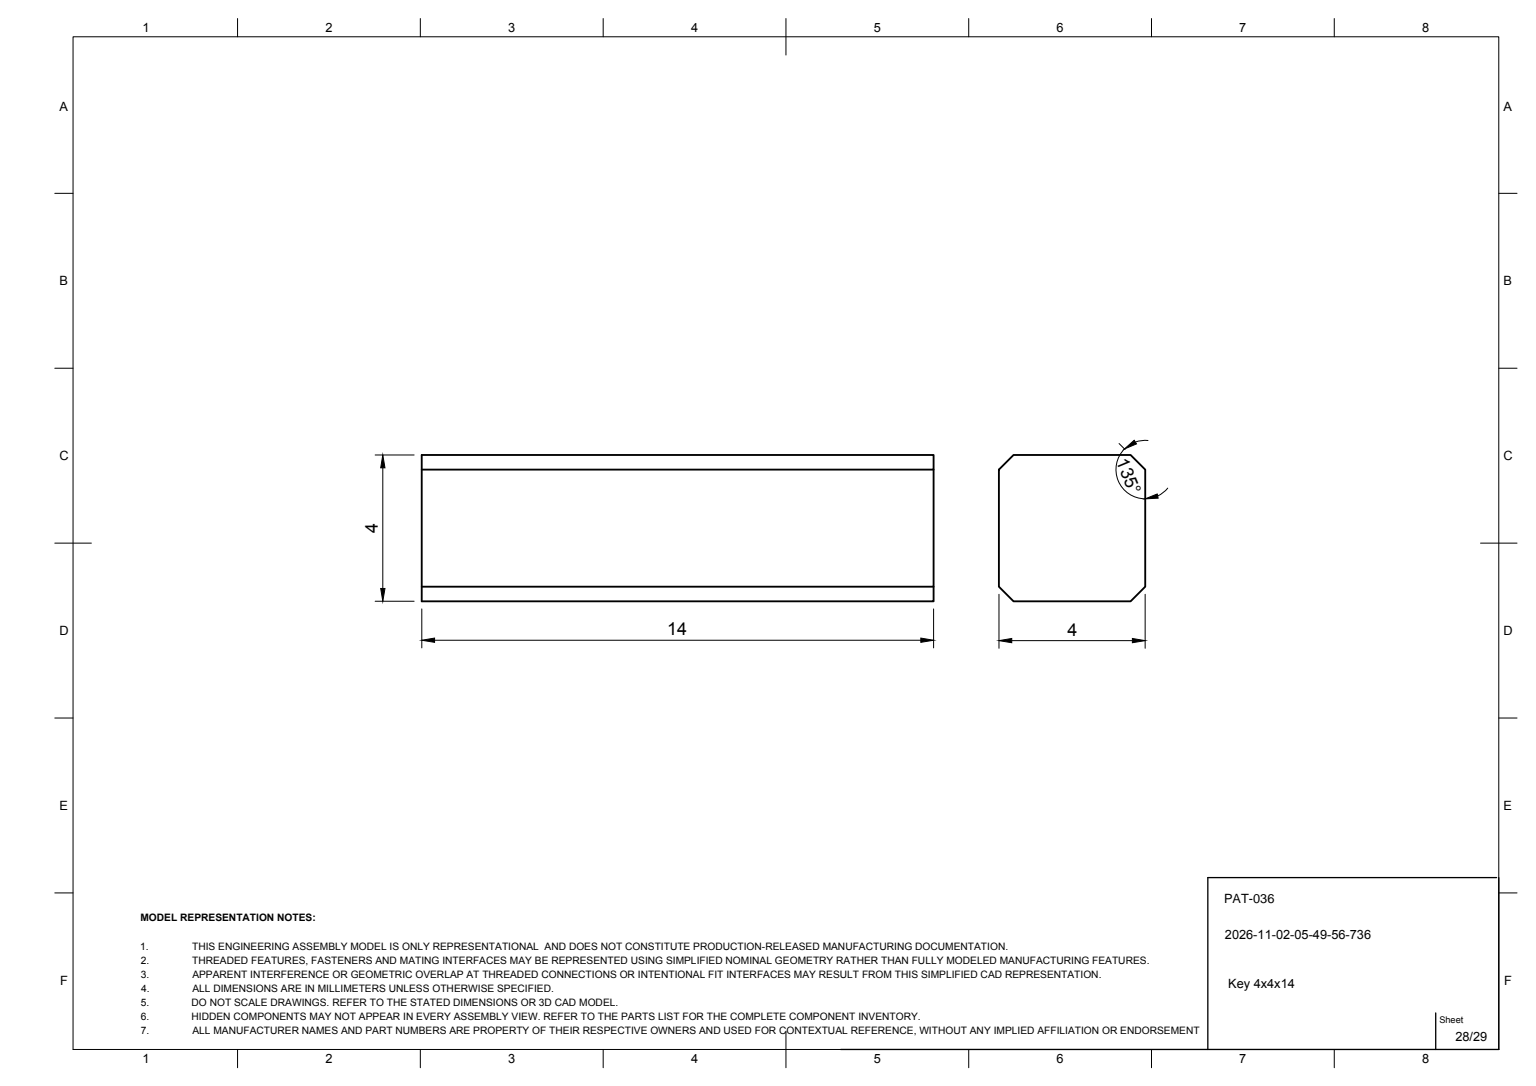
ISO-10303-21;
HEADER;
/* Generated by software containing ST-Developer
 * from STEP Tools, Inc. (www.steptools.com) 
 */

FILE_DESCRIPTION(
/* description */ ('Flange-mounted spindle'),
/* implementation_level */ '2;1');

FILE_NAME(
/* name */ 'Key 4x4x14.step',
/* time_stamp */ '2026-10-27T10:49:51-07:00',
/* author */ (''),
/* organization */ (''),
/* preprocessor_version */ 'ST-DEVELOPER v20.2',
/* originating_system */ 'Autodesk Translation Framework v15.17.0.0',
/* authorisation */ '');

FILE_SCHEMA (('AUTOMOTIVE_DESIGN { 1 0 10303 214 3 1 1 }'));
ENDSEC;

DATA;
#10=MECHANICAL_DESIGN_GEOMETRIC_PRESENTATION_REPRESENTATION('',(#360),#11764);
#305=SHAPE_REPRESENTATION_RELATIONSHIP('SRR','None',#11903,#332);
#332=ADVANCED_BREP_SHAPE_REPRESENTATION('',(#386),#11758);
#360=STYLED_ITEM('',(#12099),#386);
#386=MANIFOLD_SOLID_BREP('Body1',#6154);
#624=PLANE('',#7074);
#625=PLANE('',#7075);
#626=PLANE('',#7076);
#627=PLANE('',#7077);
#628=PLANE('',#7078);
#629=PLANE('',#7079);
#630=PLANE('',#7080);
#631=PLANE('',#7081);
#632=PLANE('',#7082);
#633=PLANE('',#7083);
#955=FACE_OUTER_BOUND('',#1409,.T.);
#956=FACE_OUTER_BOUND('',#1410,.T.);
#957=FACE_OUTER_BOUND('',#1411,.T.);
#958=FACE_OUTER_BOUND('',#1412,.T.);
#959=FACE_OUTER_BOUND('',#1413,.T.);
#960=FACE_OUTER_BOUND('',#1414,.T.);
#961=FACE_OUTER_BOUND('',#1415,.T.);
#962=FACE_OUTER_BOUND('',#1416,.T.);
#963=FACE_OUTER_BOUND('',#1417,.T.);
#964=FACE_OUTER_BOUND('',#1418,.T.);
#1409=EDGE_LOOP('',(#5353,#5354,#5355,#5356,#5357,#5358,#5359,#5360));
#1410=EDGE_LOOP('',(#5361,#5362,#5363,#5364));
#1411=EDGE_LOOP('',(#5365,#5366,#5367,#5368));
#1412=EDGE_LOOP('',(#5369,#5370,#5371,#5372));
#1413=EDGE_LOOP('',(#5373,#5374,#5375,#5376));
#1414=EDGE_LOOP('',(#5377,#5378,#5379,#5380,#5381,#5382,#5383,#5384));
#1415=EDGE_LOOP('',(#5385,#5386,#5387,#5388));
#1416=EDGE_LOOP('',(#5389,#5390,#5391,#5392));
#1417=EDGE_LOOP('',(#5393,#5394,#5395,#5396));
#1418=EDGE_LOOP('',(#5397,#5398,#5399,#5400));
#1797=LINE('',#11342,#2219);
#1798=LINE('',#11344,#2220);
#1799=LINE('',#11346,#2221);
#1800=LINE('',#11348,#2222);
#1801=LINE('',#11350,#2223);
#1802=LINE('',#11352,#2224);
#1803=LINE('',#11354,#2225);
#1804=LINE('',#11355,#2226);
#1805=LINE('',#11358,#2227);
#1806=LINE('',#11360,#2228);
#1807=LINE('',#11361,#2229);
#1808=LINE('',#11364,#2230);
#1809=LINE('',#11365,#2231);
#1810=LINE('',#11368,#2232);
#1811=LINE('',#11369,#2233);
#1812=LINE('',#11372,#2234);
#1813=LINE('',#11373,#2235);
#1814=LINE('',#11376,#2236);
#1815=LINE('',#11378,#2237);
#1816=LINE('',#11380,#2238);
#1817=LINE('',#11381,#2239);
#1818=LINE('',#11383,#2240);
#1819=LINE('',#11385,#2241);
#1820=LINE('',#11387,#2242);
#2219=VECTOR('',#8758,1.);
#2220=VECTOR('',#8759,1.);
#2221=VECTOR('',#8760,1.);
#2222=VECTOR('',#8761,1.);
#2223=VECTOR('',#8762,1.);
#2224=VECTOR('',#8763,1.);
#2225=VECTOR('',#8764,1.);
#2226=VECTOR('',#8765,1.);
#2227=VECTOR('',#8768,1.);
#2228=VECTOR('',#8769,1.);
#2229=VECTOR('',#8770,1.);
#2230=VECTOR('',#8773,1.);
#2231=VECTOR('',#8774,1.);
#2232=VECTOR('',#8777,1.);
#2233=VECTOR('',#8778,1.);
#2234=VECTOR('',#8781,1.);
#2235=VECTOR('',#8782,1.);
#2236=VECTOR('',#8785,1.);
#2237=VECTOR('',#8786,1.);
#2238=VECTOR('',#8787,1.);
#2239=VECTOR('',#8788,1.);
#2240=VECTOR('',#8791,1.);
#2241=VECTOR('',#8794,1.);
#2242=VECTOR('',#8797,1.);
#3107=VERTEX_POINT('',#11340);
#3108=VERTEX_POINT('',#11341);
#3109=VERTEX_POINT('',#11343);
#3110=VERTEX_POINT('',#11345);
#3111=VERTEX_POINT('',#11347);
#3112=VERTEX_POINT('',#11349);
#3113=VERTEX_POINT('',#11351);
#3114=VERTEX_POINT('',#11353);
#3115=VERTEX_POINT('',#11357);
#3116=VERTEX_POINT('',#11359);
#3117=VERTEX_POINT('',#11363);
#3118=VERTEX_POINT('',#11367);
#3119=VERTEX_POINT('',#11371);
#3120=VERTEX_POINT('',#11375);
#3121=VERTEX_POINT('',#11377);
#3122=VERTEX_POINT('',#11379);
#3869=EDGE_CURVE('',#3107,#3108,#1797,.T.);
#3870=EDGE_CURVE('',#3109,#3107,#1798,.T.);
#3871=EDGE_CURVE('',#3110,#3109,#1799,.T.);
#3872=EDGE_CURVE('',#3111,#3110,#1800,.T.);
#3873=EDGE_CURVE('',#3112,#3111,#1801,.T.);
#3874=EDGE_CURVE('',#3113,#3112,#1802,.T.);
#3875=EDGE_CURVE('',#3114,#3113,#1803,.T.);
#3876=EDGE_CURVE('',#3108,#3114,#1804,.T.);
#3877=EDGE_CURVE('',#3111,#3115,#1805,.T.);
#3878=EDGE_CURVE('',#3115,#3116,#1806,.T.);
#3879=EDGE_CURVE('',#3116,#3112,#1807,.T.);
#3880=EDGE_CURVE('',#3117,#3110,#1808,.T.);
#3881=EDGE_CURVE('',#3117,#3115,#1809,.T.);
#3882=EDGE_CURVE('',#3109,#3118,#1810,.T.);
#3883=EDGE_CURVE('',#3118,#3117,#1811,.T.);
#3884=EDGE_CURVE('',#3119,#3107,#1812,.T.);
#3885=EDGE_CURVE('',#3119,#3118,#1813,.T.);
#3886=EDGE_CURVE('',#3120,#3119,#1814,.T.);
#3887=EDGE_CURVE('',#3121,#3120,#1815,.T.);
#3888=EDGE_CURVE('',#3122,#3121,#1816,.T.);
#3889=EDGE_CURVE('',#3116,#3122,#1817,.T.);
#3890=EDGE_CURVE('',#3108,#3120,#1818,.T.);
#3891=EDGE_CURVE('',#3121,#3114,#1819,.T.);
#3892=EDGE_CURVE('',#3113,#3122,#1820,.T.);
#5353=ORIENTED_EDGE('',*,*,#3869,.F.);
#5354=ORIENTED_EDGE('',*,*,#3870,.F.);
#5355=ORIENTED_EDGE('',*,*,#3871,.F.);
#5356=ORIENTED_EDGE('',*,*,#3872,.F.);
#5357=ORIENTED_EDGE('',*,*,#3873,.F.);
#5358=ORIENTED_EDGE('',*,*,#3874,.F.);
#5359=ORIENTED_EDGE('',*,*,#3875,.F.);
#5360=ORIENTED_EDGE('',*,*,#3876,.F.);
#5361=ORIENTED_EDGE('',*,*,#3873,.T.);
#5362=ORIENTED_EDGE('',*,*,#3877,.T.);
#5363=ORIENTED_EDGE('',*,*,#3878,.T.);
#5364=ORIENTED_EDGE('',*,*,#3879,.T.);
#5365=ORIENTED_EDGE('',*,*,#3872,.T.);
#5366=ORIENTED_EDGE('',*,*,#3880,.F.);
#5367=ORIENTED_EDGE('',*,*,#3881,.T.);
#5368=ORIENTED_EDGE('',*,*,#3877,.F.);
#5369=ORIENTED_EDGE('',*,*,#3871,.T.);
#5370=ORIENTED_EDGE('',*,*,#3882,.T.);
#5371=ORIENTED_EDGE('',*,*,#3883,.T.);
#5372=ORIENTED_EDGE('',*,*,#3880,.T.);
#5373=ORIENTED_EDGE('',*,*,#3870,.T.);
#5374=ORIENTED_EDGE('',*,*,#3884,.F.);
#5375=ORIENTED_EDGE('',*,*,#3885,.T.);
#5376=ORIENTED_EDGE('',*,*,#3882,.F.);
#5377=ORIENTED_EDGE('',*,*,#3878,.F.);
#5378=ORIENTED_EDGE('',*,*,#3881,.F.);
#5379=ORIENTED_EDGE('',*,*,#3883,.F.);
#5380=ORIENTED_EDGE('',*,*,#3885,.F.);
#5381=ORIENTED_EDGE('',*,*,#3886,.F.);
#5382=ORIENTED_EDGE('',*,*,#3887,.F.);
#5383=ORIENTED_EDGE('',*,*,#3888,.F.);
#5384=ORIENTED_EDGE('',*,*,#3889,.F.);
#5385=ORIENTED_EDGE('',*,*,#3869,.T.);
#5386=ORIENTED_EDGE('',*,*,#3890,.T.);
#5387=ORIENTED_EDGE('',*,*,#3886,.T.);
#5388=ORIENTED_EDGE('',*,*,#3884,.T.);
#5389=ORIENTED_EDGE('',*,*,#3876,.T.);
#5390=ORIENTED_EDGE('',*,*,#3891,.F.);
#5391=ORIENTED_EDGE('',*,*,#3887,.T.);
#5392=ORIENTED_EDGE('',*,*,#3890,.F.);
#5393=ORIENTED_EDGE('',*,*,#3875,.T.);
#5394=ORIENTED_EDGE('',*,*,#3892,.T.);
#5395=ORIENTED_EDGE('',*,*,#3888,.T.);
#5396=ORIENTED_EDGE('',*,*,#3891,.T.);
#5397=ORIENTED_EDGE('',*,*,#3874,.T.);
#5398=ORIENTED_EDGE('',*,*,#3879,.F.);
#5399=ORIENTED_EDGE('',*,*,#3889,.T.);
#5400=ORIENTED_EDGE('',*,*,#3892,.F.);
#6066=ADVANCED_FACE('',(#955),#624,.T.);
#6067=ADVANCED_FACE('',(#956),#625,.T.);
#6068=ADVANCED_FACE('',(#957),#626,.T.);
#6069=ADVANCED_FACE('',(#958),#627,.T.);
#6070=ADVANCED_FACE('',(#959),#628,.T.);
#6071=ADVANCED_FACE('',(#960),#629,.F.);
#6072=ADVANCED_FACE('',(#961),#630,.T.);
#6073=ADVANCED_FACE('',(#962),#631,.T.);
#6074=ADVANCED_FACE('',(#963),#632,.T.);
#6075=ADVANCED_FACE('',(#964),#633,.F.);
#6154=CLOSED_SHELL('',(#6066,#6067,#6068,#6069,#6070,#6071,#6072,#6073,
#6074,#6075));
#7073=AXIS2_PLACEMENT_3D('',#11338,#8754,#8755);
#7074=AXIS2_PLACEMENT_3D('',#11339,#8756,#8757);
#7075=AXIS2_PLACEMENT_3D('',#11356,#8766,#8767);
#7076=AXIS2_PLACEMENT_3D('',#11362,#8771,#8772);
#7077=AXIS2_PLACEMENT_3D('',#11366,#8775,#8776);
#7078=AXIS2_PLACEMENT_3D('',#11370,#8779,#8780);
#7079=AXIS2_PLACEMENT_3D('',#11374,#8783,#8784);
#7080=AXIS2_PLACEMENT_3D('',#11382,#8789,#8790);
#7081=AXIS2_PLACEMENT_3D('',#11384,#8792,#8793);
#7082=AXIS2_PLACEMENT_3D('',#11386,#8795,#8796);
#7083=AXIS2_PLACEMENT_3D('',#11388,#8798,#8799);
#8754=DIRECTION('axis',(0.,0.,1.));
#8755=DIRECTION('refdir',(1.,0.,0.));
#8756=DIRECTION('center_axis',(1.,0.,0.));
#8757=DIRECTION('ref_axis',(0.,0.,-1.));
#8758=DIRECTION('',(0.,0.707106781186547,-0.707106781186548));
#8759=DIRECTION('',(0.,1.,0.));
#8760=DIRECTION('',(0.,0.707106781186547,0.707106781186548));
#8761=DIRECTION('',(0.,0.,1.));
#8762=DIRECTION('',(0.,-0.707106781186548,0.707106781186548));
#8763=DIRECTION('',(0.,-1.,0.));
#8764=DIRECTION('',(0.,-0.707106781186548,-0.707106781186548));
#8765=DIRECTION('',(0.,0.,-1.));
#8766=DIRECTION('center_axis',(0.,-0.707106781186548,-0.707106781186548));
#8767=DIRECTION('ref_axis',(-1.,0.,0.));
#8768=DIRECTION('',(-1.,0.,0.));
#8769=DIRECTION('',(0.,0.707106781186548,-0.707106781186548));
#8770=DIRECTION('',(1.,0.,0.));
#8771=DIRECTION('center_axis',(0.,-1.,0.));
#8772=DIRECTION('ref_axis',(1.,0.,0.));
#8773=DIRECTION('',(1.,0.,0.));
#8774=DIRECTION('',(0.,0.,-1.));
#8775=DIRECTION('center_axis',(0.,-0.707106781186548,0.707106781186547));
#8776=DIRECTION('ref_axis',(1.,0.,0.));
#8777=DIRECTION('',(-1.,0.,0.));
#8778=DIRECTION('',(0.,-0.707106781186547,-0.707106781186548));
#8779=DIRECTION('center_axis',(0.,0.,1.));
#8780=DIRECTION('ref_axis',(1.,0.,0.));
#8781=DIRECTION('',(1.,0.,0.));
#8782=DIRECTION('',(0.,-1.,0.));
#8783=DIRECTION('center_axis',(1.,0.,0.));
#8784=DIRECTION('ref_axis',(0.,0.,-1.));
#8785=DIRECTION('',(0.,-0.707106781186547,0.707106781186548));
#8786=DIRECTION('',(0.,0.,1.));
#8787=DIRECTION('',(0.,0.707106781186548,0.707106781186548));
#8788=DIRECTION('',(0.,1.,0.));
#8789=DIRECTION('center_axis',(0.,0.707106781186548,0.707106781186547));
#8790=DIRECTION('ref_axis',(1.,0.,0.));
#8791=DIRECTION('',(-1.,0.,0.));
#8792=DIRECTION('center_axis',(0.,1.,0.));
#8793=DIRECTION('ref_axis',(-1.,0.,0.));
#8794=DIRECTION('',(1.,0.,0.));
#8795=DIRECTION('center_axis',(0.,0.707106781186548,-0.707106781186548));
#8796=DIRECTION('ref_axis',(-1.,0.,0.));
#8797=DIRECTION('',(-1.,0.,0.));
#8798=DIRECTION('center_axis',(0.,0.,1.));
#8799=DIRECTION('ref_axis',(1.,0.,0.));
#11338=CARTESIAN_POINT('',(0.,0.,0.));
#11339=CARTESIAN_POINT('Origin',(0.7,0.,0.25));
#11340=CARTESIAN_POINT('',(0.7,0.16,0.4));
#11341=CARTESIAN_POINT('',(0.7,0.2,0.36));
#11342=CARTESIAN_POINT('',(0.7,0.1675,0.3925));
#11343=CARTESIAN_POINT('',(0.7,-0.16,0.4));
#11344=CARTESIAN_POINT('',(0.7,0.,0.4));
#11345=CARTESIAN_POINT('',(0.7,-0.2,0.36));
#11346=CARTESIAN_POINT('',(0.7,-0.1675,0.3925));
#11347=CARTESIAN_POINT('',(0.7,-0.2,0.04));
#11348=CARTESIAN_POINT('',(0.7,-0.2,0.125));
#11349=CARTESIAN_POINT('',(0.7,-0.16,0.));
#11350=CARTESIAN_POINT('',(0.7,-0.1925,0.0325));
#11351=CARTESIAN_POINT('',(0.7,0.16,0.));
#11352=CARTESIAN_POINT('',(0.7,0.,0.));
#11353=CARTESIAN_POINT('',(0.7,0.2,0.04));
#11354=CARTESIAN_POINT('',(0.7,0.1925,0.0325));
#11355=CARTESIAN_POINT('',(0.7,0.2,0.125));
#11356=CARTESIAN_POINT('Origin',(-0.4,-0.18,0.02));
#11357=CARTESIAN_POINT('',(-0.7,-0.2,0.04));
#11358=CARTESIAN_POINT('',(-0.4,-0.2,0.04));
#11359=CARTESIAN_POINT('',(-0.7,-0.16,0.));
#11360=CARTESIAN_POINT('',(-0.7,-0.1925,0.0325));
#11361=CARTESIAN_POINT('',(-0.4,-0.16,0.));
#11362=CARTESIAN_POINT('Origin',(-0.8,-0.2,0.));
#11363=CARTESIAN_POINT('',(-0.7,-0.2,0.36));
#11364=CARTESIAN_POINT('',(-0.4,-0.2,0.36));
#11365=CARTESIAN_POINT('',(-0.7,-0.2,0.125));
#11366=CARTESIAN_POINT('Origin',(-0.4,-0.18,0.38));
#11367=CARTESIAN_POINT('',(-0.7,-0.16,0.4));
#11368=CARTESIAN_POINT('',(-0.4,-0.16,0.4));
#11369=CARTESIAN_POINT('',(-0.7,-0.1675,0.3925));
#11370=CARTESIAN_POINT('Origin',(0.,0.,0.4));
#11371=CARTESIAN_POINT('',(-0.7,0.16,0.4));
#11372=CARTESIAN_POINT('',(0.4,0.16,0.4));
#11373=CARTESIAN_POINT('',(-0.7,0.,0.4));
#11374=CARTESIAN_POINT('Origin',(-0.7,0.,0.25));
#11375=CARTESIAN_POINT('',(-0.7,0.2,0.36));
#11376=CARTESIAN_POINT('',(-0.7,0.1675,0.3925));
#11377=CARTESIAN_POINT('',(-0.7,0.2,0.04));
#11378=CARTESIAN_POINT('',(-0.7,0.2,0.125));
#11379=CARTESIAN_POINT('',(-0.7,0.16,0.));
#11380=CARTESIAN_POINT('',(-0.7,0.1925,0.0325));
#11381=CARTESIAN_POINT('',(-0.7,0.,0.));
#11382=CARTESIAN_POINT('Origin',(0.4,0.18,0.38));
#11383=CARTESIAN_POINT('',(0.4,0.2,0.36));
#11384=CARTESIAN_POINT('Origin',(0.8,0.2,0.));
#11385=CARTESIAN_POINT('',(0.4,0.2,0.04));
#11386=CARTESIAN_POINT('Origin',(0.4,0.18,0.02));
#11387=CARTESIAN_POINT('',(0.4,0.16,0.));
#11388=CARTESIAN_POINT('Origin',(0.,0.,0.));
#11726=UNCERTAINTY_MEASURE_WITH_UNIT(LENGTH_MEASURE(0.001),#11765,
'DISTANCE_ACCURACY_VALUE',
'Maximum model space distance between geometric entities at asserted c
onnectivities');
#11732=UNCERTAINTY_MEASURE_WITH_UNIT(LENGTH_MEASURE(0.001),#11765,
'DISTANCE_ACCURACY_VALUE',
'Maximum model space distance between geometric entities at asserted c
onnectivities');
#11758=(
GEOMETRIC_REPRESENTATION_CONTEXT(3)
GLOBAL_UNCERTAINTY_ASSIGNED_CONTEXT((#11726))
GLOBAL_UNIT_ASSIGNED_CONTEXT((#11765,#11767,#11768))
REPRESENTATION_CONTEXT('','3D')
);
#11764=(
GEOMETRIC_REPRESENTATION_CONTEXT(3)
GLOBAL_UNCERTAINTY_ASSIGNED_CONTEXT((#11732))
GLOBAL_UNIT_ASSIGNED_CONTEXT((#11765,#11767,#11768))
REPRESENTATION_CONTEXT('','3D')
);
#11765=(
LENGTH_UNIT()
NAMED_UNIT(*)
SI_UNIT(.CENTI.,.METRE.)
);
#11767=(
NAMED_UNIT(*)
PLANE_ANGLE_UNIT()
SI_UNIT($,.RADIAN.)
);
#11768=(
NAMED_UNIT(*)
SI_UNIT($,.STERADIAN.)
SOLID_ANGLE_UNIT()
);
#11794=SHAPE_DEFINITION_REPRESENTATION(#11827,#11903);
#11827=PRODUCT_DEFINITION_SHAPE('',$,#11935);
#11903=SHAPE_REPRESENTATION('',(#7073),#11758);
#11909=PRODUCT_DEFINITION_CONTEXT('part definition',#12004,'design');
#11935=PRODUCT_DEFINITION('Key 4x4x14','Key 4x4x14',#11966,#11909);
#11966=PRODUCT_DEFINITION_FORMATION('',$,#12031);
#12004=APPLICATION_CONTEXT(
'Core Data for Automotive Mechanical Design Process');
#12005=PRODUCT_CONTEXT('part definition',#12004,'mechanical');
#12031=PRODUCT('Key 4x4x14','Key 4x4x14','Key 4x4x14',(#12005));
#12093=COLOUR_RGB('Grey',0.48,0.52,0.57);
#12094=FILL_AREA_STYLE_COLOUR('',#12093);
#12095=FILL_AREA_STYLE('',(#12094));
#12096=SURFACE_STYLE_FILL_AREA(#12095);
#12097=SURFACE_SIDE_STYLE('',(#12096));
#12098=SURFACE_STYLE_USAGE(.BOTH.,#12097);
#12099=PRESENTATION_STYLE_ASSIGNMENT((#12098));
ENDSEC;
END-ISO-10303-21;
